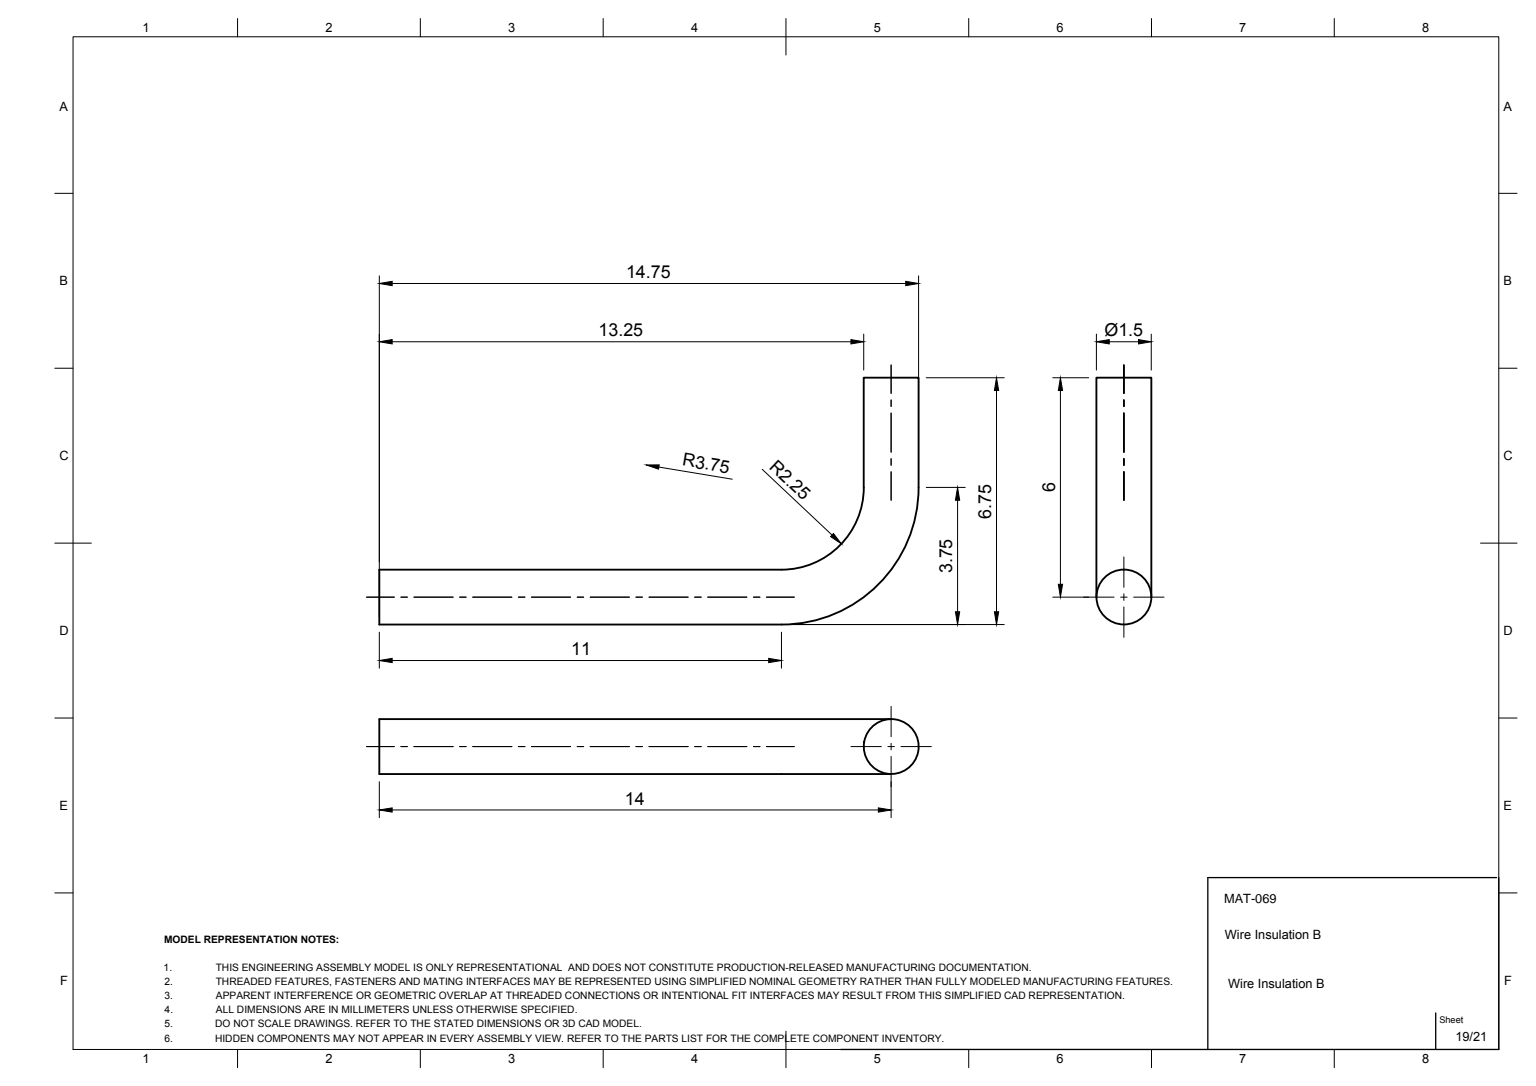
ISO-10303-21;
HEADER;
/* Generated by software containing ST-Developer
 * from STEP Tools, Inc. (www.steptools.com) 
 */

FILE_DESCRIPTION(
/* description */ ('CAx-IF Rec.Pracs.---Representation and Presentation of Product Manufa
cturing Information (PMI)---4.0---2014-10-13'),
/* implementation_level */ '2;1');

FILE_NAME(
/* name */ 'Wire Insulation B.step',
/* time_stamp */ '2026-10-24T15:08:39-07:00',
/* author */ (''),
/* organization */ (''),
/* preprocessor_version */ 'ST-DEVELOPER v20.2',
/* originating_system */ 'Autodesk Translation Framework v15.17.0.0',
/* authorisation */ '');

FILE_SCHEMA (('AP242_MANAGED_MODEL_BASED_3D_ENGINEERING_MIM_LF { 1 0 10303 442 2 1 4 }'));
ENDSEC;

DATA;
#10=MECHANICAL_DESIGN_GEOMETRIC_PRESENTATION_REPRESENTATION('',(#837),#50081);
#778=TOROIDAL_SURFACE('',#10973,0.003,0.00075);
#797=SHAPE_REPRESENTATION_RELATIONSHIP('SRR','None',#50165,#817);
#817=ADVANCED_BREP_SHAPE_REPRESENTATION('',(#857),#50078);
#837=STYLED_ITEM('',(#50259),#857);
#857=MANIFOLD_SOLID_BREP('Body1',#9882);
#1095=PLANE('',#10967);
#1096=PLANE('',#10978);
#1620=FACE_OUTER_BOUND('',#2218,.T.);
#1621=FACE_OUTER_BOUND('',#2219,.T.);
#1622=FACE_OUTER_BOUND('',#2220,.T.);
#1623=FACE_OUTER_BOUND('',#2221,.T.);
#1624=FACE_OUTER_BOUND('',#2222,.T.);
#2218=EDGE_LOOP('',(#9042));
#2219=EDGE_LOOP('',(#9043,#9044,#9045,#9046,#9047));
#2220=EDGE_LOOP('',(#9048,#9049,#9050,#9051,#9052,#9053));
#2221=EDGE_LOOP('',(#9054,#9055,#9056,#9057,#9058));
#2222=EDGE_LOOP('',(#9059));
#2811=LINE('',#49266,#3389);
#2812=LINE('',#49277,#3390);
#3389=VECTOR('',#13333,0.00075);
#3390=VECTOR('',#13348,0.00075);
#3747=CIRCLE('',#10968,0.00075000000001);
#3748=CIRCLE('',#10970,0.00075000000001);
#3749=CIRCLE('',#10971,0.00075000000001);
#3750=CIRCLE('',#10972,0.00075000000001);
#3751=CIRCLE('',#10974,0.00225);
#3752=CIRCLE('',#10975,0.00075000000001);
#3753=CIRCLE('',#10976,0.00075000000001);
#4731=VERTEX_POINT('',#49260);
#4732=VERTEX_POINT('',#49263);
#4733=VERTEX_POINT('',#49265);
#4734=VERTEX_POINT('',#49267);
#4735=VERTEX_POINT('',#49271);
#4736=VERTEX_POINT('',#49273);
#6174=EDGE_CURVE('',#4731,#4731,#3747,.T.);
#6175=EDGE_CURVE('',#4732,#4732,#3748,.T.);
#6176=EDGE_CURVE('',#4732,#4733,#2811,.T.);
#6177=EDGE_CURVE('',#4733,#4734,#3749,.T.);
#6178=EDGE_CURVE('',#4734,#4733,#3750,.T.);
#6179=EDGE_CURVE('',#4734,#4735,#3751,.T.);
#6180=EDGE_CURVE('',#4735,#4736,#3752,.T.);
#6181=EDGE_CURVE('',#4736,#4735,#3753,.T.);
#6182=EDGE_CURVE('',#4736,#4731,#2812,.T.);
#9042=ORIENTED_EDGE('',*,*,#6174,.F.);
#9043=ORIENTED_EDGE('',*,*,#6175,.F.);
#9044=ORIENTED_EDGE('',*,*,#6176,.T.);
#9045=ORIENTED_EDGE('',*,*,#6177,.T.);
#9046=ORIENTED_EDGE('',*,*,#6178,.T.);
#9047=ORIENTED_EDGE('',*,*,#6176,.F.);
#9048=ORIENTED_EDGE('',*,*,#6178,.F.);
#9049=ORIENTED_EDGE('',*,*,#6179,.T.);
#9050=ORIENTED_EDGE('',*,*,#6180,.T.);
#9051=ORIENTED_EDGE('',*,*,#6181,.T.);
#9052=ORIENTED_EDGE('',*,*,#6179,.F.);
#9053=ORIENTED_EDGE('',*,*,#6177,.F.);
#9054=ORIENTED_EDGE('',*,*,#6181,.F.);
#9055=ORIENTED_EDGE('',*,*,#6182,.T.);
#9056=ORIENTED_EDGE('',*,*,#6174,.T.);
#9057=ORIENTED_EDGE('',*,*,#6182,.F.);
#9058=ORIENTED_EDGE('',*,*,#6180,.F.);
#9059=ORIENTED_EDGE('',*,*,#6175,.T.);
#9315=CYLINDRICAL_SURFACE('',#10969,0.00075);
#9316=CYLINDRICAL_SURFACE('',#10977,0.00075);
#9842=ADVANCED_FACE('',(#1620),#1095,.F.);
#9843=ADVANCED_FACE('',(#1621),#9315,.T.);
#9844=ADVANCED_FACE('',(#1622),#778,.T.);
#9845=ADVANCED_FACE('',(#1623),#9316,.T.);
#9846=ADVANCED_FACE('',(#1624),#1096,.T.);
#9882=CLOSED_SHELL('',(#9842,#9843,#9844,#9845,#9846));
#10966=AXIS2_PLACEMENT_3D('',#49258,#13323,#13324);
#10967=AXIS2_PLACEMENT_3D('',#49259,#13325,#13326);
#10968=AXIS2_PLACEMENT_3D('',#49261,#13327,#13328);
#10969=AXIS2_PLACEMENT_3D('',#49262,#13329,#13330);
#10970=AXIS2_PLACEMENT_3D('',#49264,#13331,#13332);
#10971=AXIS2_PLACEMENT_3D('',#49268,#13334,#13335);
#10972=AXIS2_PLACEMENT_3D('',#49269,#13336,#13337);
#10973=AXIS2_PLACEMENT_3D('',#49270,#13338,#13339);
#10974=AXIS2_PLACEMENT_3D('',#49272,#13340,#13341);
#10975=AXIS2_PLACEMENT_3D('',#49274,#13342,#13343);
#10976=AXIS2_PLACEMENT_3D('',#49275,#13344,#13345);
#10977=AXIS2_PLACEMENT_3D('',#49276,#13346,#13347);
#10978=AXIS2_PLACEMENT_3D('',#49278,#13349,#13350);
#13323=DIRECTION('axis',(0.,0.,1.));
#13324=DIRECTION('refdir',(1.,0.,0.));
#13325=DIRECTION('center_axis',(0.984807753012209,-0.173648177666927,-6.9026791896102E-15));
#13326=DIRECTION('ref_axis',(6.74488507274914E-15,-1.49880108324396E-15,
1.));
#13327=DIRECTION('center_axis',(0.984807753012209,-0.173648177666927,-6.9026791896102E-15));
#13328=DIRECTION('ref_axis',(-0.173648177666927,-0.984807753012209,-1.41609297436625E-15));
#13329=DIRECTION('center_axis',(-6.74488507274914E-15,1.49880108324396E-15,
-1.));
#13330=DIRECTION('ref_axis',(-0.173648177666927,-0.984807753012209,-3.04793925546002E-16));
#13331=DIRECTION('center_axis',(1.31243041282465E-11,-2.31385942497016E-12,
-1.));
#13332=DIRECTION('ref_axis',(-0.173648177666927,-0.984807753012209,-3.04793925546223E-16));
#13333=DIRECTION('',(6.74488507274914E-15,-1.49880108324396E-15,1.));
#13334=DIRECTION('center_axis',(1.31243041282465E-11,-2.31385942497016E-12,
-1.));
#13335=DIRECTION('ref_axis',(-0.173648177666927,-0.984807753012209,-3.04793925546223E-16));
#13336=DIRECTION('center_axis',(1.31243041282465E-11,-2.31385942497016E-12,
-1.));
#13337=DIRECTION('ref_axis',(-0.173648177666927,-0.984807753012209,-3.04793925546223E-16));
#13338=DIRECTION('center_axis',(0.173648177666927,0.984807753012209,1.41609297436625E-15));
#13339=DIRECTION('ref_axis',(-6.47630097698008E-15,1.85037170770859E-15,
-1.));
#13340=DIRECTION('center_axis',(-0.173648177666927,-0.984807753012209,-1.41609297436625E-15));
#13341=DIRECTION('ref_axis',(-6.31282311555423E-15,2.55105953078819E-15,
-1.));
#13342=DIRECTION('center_axis',(0.984807753012209,-0.173648177666927,-6.9026791896102E-15));
#13343=DIRECTION('ref_axis',(-0.173648177666927,-0.984807753012209,-1.41609297436625E-15));
#13344=DIRECTION('center_axis',(0.984807753012209,-0.173648177666927,-6.9026791896102E-15));
#13345=DIRECTION('ref_axis',(-0.173648177666927,-0.984807753012209,-1.41609297436625E-15));
#13346=DIRECTION('center_axis',(0.984807753012209,-0.173648177666927,-6.9026791896102E-15));
#13347=DIRECTION('ref_axis',(-0.173648177666927,-0.984807753012209,-1.41609297436625E-15));
#13348=DIRECTION('',(-0.984807753012209,0.173648177666927,6.9026791896102E-15));
#13349=DIRECTION('center_axis',(-6.46591174117934E-15,1.44961055799008E-15,
-1.));
#13350=DIRECTION('ref_axis',(-0.173648177666927,-0.984807753012209,-3.04793925546006E-16));
#49258=CARTESIAN_POINT('',(0.,0.,0.));
#49259=CARTESIAN_POINT('Origin',(-0.0205477808086712,-0.0363249115320537,
0.0038241467581455));
#49260=CARTESIAN_POINT('',(-0.0204175446754309,-0.0355863057172927,0.00382414675814549));
#49261=CARTESIAN_POINT('Origin',(-0.0205477808086811,-0.0363249115320519,
0.0038241467581555));
#49262=CARTESIAN_POINT('Origin',(-0.00676047226650036,-0.0387559860193906,
0.000824146758145397));
#49263=CARTESIAN_POINT('',(-0.00663023613325018,-0.0380173802046314,-0.00217585328655808));
#49264=CARTESIAN_POINT('Origin',(-0.00676047226651023,-0.0387559860193889,
-0.00217585328654808));
#49265=CARTESIAN_POINT('',(-0.00663023613325016,-0.0380173802046314,0.000824146758165397));
#49266=CARTESIAN_POINT('',(-0.00663023613325016,-0.0380173802046314,0.000824146758145397));
#49267=CARTESIAN_POINT('',(-0.0074990780812792,-0.0386257498861369,0.000824146758145402));
#49268=CARTESIAN_POINT('Origin',(-0.00676047226651021,-0.0387559860193889,
0.000824146758155397));
#49269=CARTESIAN_POINT('Origin',(-0.00676047226651021,-0.0387559860193889,
0.000824146758155397));
#49270=CARTESIAN_POINT('Origin',(-0.00971489552553699,-0.0382350414863898,
0.000824146758145418));
#49271=CARTESIAN_POINT('',(-0.00971489552554682,-0.0382350414863881,0.00307414675814542));
#49272=CARTESIAN_POINT('Origin',(-0.00971489552553699,-0.0382350414863898,
0.000824146758145418));
#49273=CARTESIAN_POINT('',(-0.00958465939229661,-0.0374964356716289,0.00382414675814542));
#49274=CARTESIAN_POINT('Origin',(-0.00971489552554682,-0.0382350414863881,
0.00382414675815542));
#49275=CARTESIAN_POINT('Origin',(-0.00971489552554682,-0.0382350414863881,
0.00382414675815542));
#49276=CARTESIAN_POINT('Origin',(-0.0244870118207201,-0.0356303188213859,
0.00382414675814552));
#49277=CARTESIAN_POINT('',(-0.0243567756874699,-0.0348917130066267,0.00382414675814552));
#49278=CARTESIAN_POINT('Origin',(-0.00676047226650038,-0.0387559860193906,
-0.00217585328655808));
#50056=UNCERTAINTY_MEASURE_WITH_UNIT(LENGTH_MEASURE(1.E-5),#50082,
'DISTANCE_ACCURACY_VALUE',
'Maximum model space distance between geometric entities at asserted c
onnectivities');
#50059=UNCERTAINTY_MEASURE_WITH_UNIT(LENGTH_MEASURE(1.E-5),#50082,
'DISTANCE_ACCURACY_VALUE',
'Maximum model space distance between geometric entities at asserted c
onnectivities');
#50078=(
GEOMETRIC_REPRESENTATION_CONTEXT(3)
GLOBAL_UNCERTAINTY_ASSIGNED_CONTEXT((#50056))
GLOBAL_UNIT_ASSIGNED_CONTEXT((#50082,#50083,#50084))
REPRESENTATION_CONTEXT('','3D')
);
#50081=(
GEOMETRIC_REPRESENTATION_CONTEXT(3)
GLOBAL_UNCERTAINTY_ASSIGNED_CONTEXT((#50059))
GLOBAL_UNIT_ASSIGNED_CONTEXT((#50082,#50083,#50084))
REPRESENTATION_CONTEXT('','3D')
);
#50082=(
LENGTH_UNIT()
NAMED_UNIT(*)
SI_UNIT($,.METRE.)
);
#50083=(
NAMED_UNIT(*)
PLANE_ANGLE_UNIT()
SI_UNIT($,.RADIAN.)
);
#50084=(
NAMED_UNIT(*)
SI_UNIT($,.STERADIAN.)
SOLID_ANGLE_UNIT()
);
#50103=SHAPE_DEFINITION_REPRESENTATION(#50124,#50165);
#50124=PRODUCT_DEFINITION_SHAPE('',$,#50187);
#50165=SHAPE_REPRESENTATION('',(#10966),#50078);
#50168=PRODUCT_DEFINITION_CONTEXT('part definition',#50233,'design');
#50187=PRODUCT_DEFINITION('Wire Insulation B','Wire Insulation B',#50208,
#50168);
#50208=PRODUCT_DEFINITION_FORMATION('',$,#50253);
#50233=APPLICATION_CONTEXT('Managed model based 3d engineering');
#50234=PRODUCT_CONTEXT('part definition',#50233,'mechanical');
#50253=PRODUCT('Wire Insulation B','Wire Insulation B','Component3',(#50234));
#50259=PRESENTATION_STYLE_ASSIGNMENT((#50266));
#50266=SURFACE_STYLE_USAGE(.BOTH.,#50273);
#50273=SURFACE_SIDE_STYLE('',(#50280));
#50280=SURFACE_STYLE_FILL_AREA(#50287);
#50287=FILL_AREA_STYLE('Opaque(246,246,243)',(#50294));
#50294=FILL_AREA_STYLE_COLOUR('Opaque(246,246,243)',#50301);
#50301=COLOUR_RGB('Opaque(246,246,243)',0.964705882352941,0.964705882352941,
0.952941176470588);
ENDSEC;
END-ISO-10303-21;
